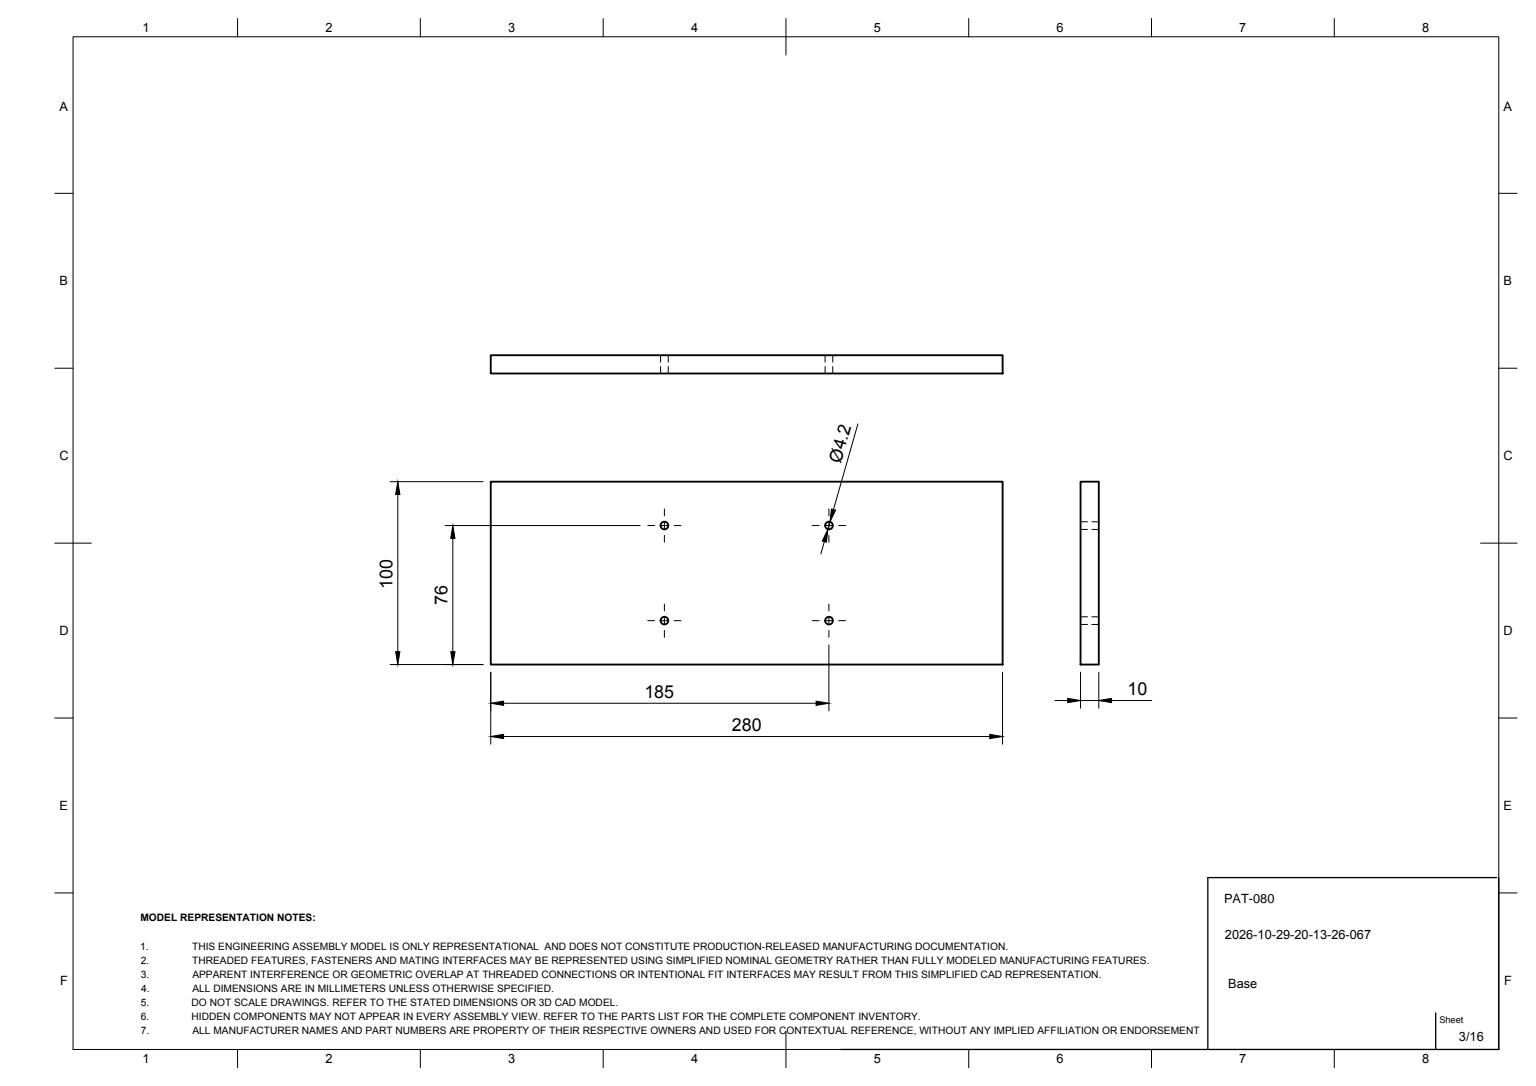
ISO-10303-21;
HEADER;
/* Generated by software containing ST-Developer
 * from STEP Tools, Inc. (www.steptools.com) 
 */

FILE_DESCRIPTION(
/* description */ ('PAT-080'),
/* implementation_level */ '2;1');

FILE_NAME(
/* name */ 'Base.step',
/* time_stamp */ '2026-10-29T20:13:47-07:00',
/* author */ (''),
/* organization */ (''),
/* preprocessor_version */ 'ST-DEVELOPER v20.2',
/* originating_system */ 'Autodesk Translation Framework v15.17.0.0',
/* authorisation */ '');

FILE_SCHEMA (('AUTOMOTIVE_DESIGN { 1 0 10303 214 3 1 1 }'));
ENDSEC;

DATA;
#10=MECHANICAL_DESIGN_GEOMETRIC_PRESENTATION_REPRESENTATION('',(#246),#6878);
#208=SHAPE_REPRESENTATION_RELATIONSHIP('SRR','None',#6964,#227);
#227=ADVANCED_BREP_SHAPE_REPRESENTATION('',(#265),#6859);
#246=STYLED_ITEM('',(#7108),#265);
#265=MANIFOLD_SOLID_BREP('Body1',#3862);
#281=FACE_BOUND('',#735,.T.);
#282=FACE_BOUND('',#736,.T.);
#283=FACE_BOUND('',#737,.T.);
#284=FACE_BOUND('',#738,.T.);
#285=FACE_BOUND('',#740,.T.);
#286=FACE_BOUND('',#741,.T.);
#287=FACE_BOUND('',#742,.T.);
#288=FACE_BOUND('',#743,.T.);
#357=PLANE('',#4108);
#358=PLANE('',#4109);
#359=PLANE('',#4110);
#360=PLANE('',#4111);
#361=PLANE('',#4112);
#362=PLANE('',#4113);
#500=FACE_OUTER_BOUND('',#726,.T.);
#501=FACE_OUTER_BOUND('',#727,.T.);
#502=FACE_OUTER_BOUND('',#728,.T.);
#503=FACE_OUTER_BOUND('',#729,.T.);
#504=FACE_OUTER_BOUND('',#730,.T.);
#505=FACE_OUTER_BOUND('',#731,.T.);
#506=FACE_OUTER_BOUND('',#732,.T.);
#507=FACE_OUTER_BOUND('',#733,.T.);
#508=FACE_OUTER_BOUND('',#734,.T.);
#509=FACE_OUTER_BOUND('',#739,.T.);
#726=EDGE_LOOP('',(#2608,#2609,#2610,#2611));
#727=EDGE_LOOP('',(#2612,#2613,#2614,#2615));
#728=EDGE_LOOP('',(#2616,#2617,#2618,#2619));
#729=EDGE_LOOP('',(#2620,#2621,#2622,#2623));
#730=EDGE_LOOP('',(#2624,#2625,#2626,#2627));
#731=EDGE_LOOP('',(#2628,#2629,#2630,#2631));
#732=EDGE_LOOP('',(#2632,#2633,#2634,#2635));
#733=EDGE_LOOP('',(#2636,#2637,#2638,#2639));
#734=EDGE_LOOP('',(#2640,#2641,#2642,#2643));
#735=EDGE_LOOP('',(#2644));
#736=EDGE_LOOP('',(#2645));
#737=EDGE_LOOP('',(#2646));
#738=EDGE_LOOP('',(#2647));
#739=EDGE_LOOP('',(#2648,#2649,#2650,#2651));
#740=EDGE_LOOP('',(#2652));
#741=EDGE_LOOP('',(#2653));
#742=EDGE_LOOP('',(#2654));
#743=EDGE_LOOP('',(#2655));
#1028=LINE('',#5735,#1343);
#1029=LINE('',#5741,#1344);
#1030=LINE('',#5747,#1345);
#1031=LINE('',#5753,#1346);
#1032=LINE('',#5758,#1347);
#1033=LINE('',#5760,#1348);
#1034=LINE('',#5762,#1349);
#1035=LINE('',#5763,#1350);
#1036=LINE('',#5766,#1351);
#1037=LINE('',#5768,#1352);
#1038=LINE('',#5769,#1353);
#1039=LINE('',#5772,#1354);
#1040=LINE('',#5774,#1355);
#1041=LINE('',#5775,#1356);
#1042=LINE('',#5777,#1357);
#1043=LINE('',#5778,#1358);
#1343=VECTOR('',#4542,0.21);
#1344=VECTOR('',#4549,0.21);
#1345=VECTOR('',#4556,0.21);
#1346=VECTOR('',#4563,0.21);
#1347=VECTOR('',#4568,1.);
#1348=VECTOR('',#4569,1.);
#1349=VECTOR('',#4570,1.);
#1350=VECTOR('',#4571,1.);
#1351=VECTOR('',#4574,1.);
#1352=VECTOR('',#4575,1.);
#1353=VECTOR('',#4576,1.);
#1354=VECTOR('',#4579,1.);
#1355=VECTOR('',#4580,1.);
#1356=VECTOR('',#4581,1.);
#1357=VECTOR('',#4584,1.);
#1358=VECTOR('',#4585,1.);
#1658=CIRCLE('',#4097,0.21);
#1659=CIRCLE('',#4098,0.21);
#1660=CIRCLE('',#4100,0.21);
#1661=CIRCLE('',#4101,0.21);
#1662=CIRCLE('',#4103,0.21);
#1663=CIRCLE('',#4104,0.21);
#1664=CIRCLE('',#4106,0.21);
#1665=CIRCLE('',#4107,0.21);
#1810=VERTEX_POINT('',#5732);
#1811=VERTEX_POINT('',#5734);
#1812=VERTEX_POINT('',#5738);
#1813=VERTEX_POINT('',#5740);
#1814=VERTEX_POINT('',#5744);
#1815=VERTEX_POINT('',#5746);
#1816=VERTEX_POINT('',#5750);
#1817=VERTEX_POINT('',#5752);
#1818=VERTEX_POINT('',#5756);
#1819=VERTEX_POINT('',#5757);
#1820=VERTEX_POINT('',#5759);
#1821=VERTEX_POINT('',#5761);
#1822=VERTEX_POINT('',#5765);
#1823=VERTEX_POINT('',#5767);
#1824=VERTEX_POINT('',#5771);
#1825=VERTEX_POINT('',#5773);
#2127=EDGE_CURVE('',#1810,#1810,#1658,.T.);
#2128=EDGE_CURVE('',#1810,#1811,#1028,.T.);
#2129=EDGE_CURVE('',#1811,#1811,#1659,.T.);
#2130=EDGE_CURVE('',#1812,#1812,#1660,.T.);
#2131=EDGE_CURVE('',#1812,#1813,#1029,.T.);
#2132=EDGE_CURVE('',#1813,#1813,#1661,.T.);
#2133=EDGE_CURVE('',#1814,#1814,#1662,.T.);
#2134=EDGE_CURVE('',#1814,#1815,#1030,.T.);
#2135=EDGE_CURVE('',#1815,#1815,#1663,.T.);
#2136=EDGE_CURVE('',#1816,#1816,#1664,.T.);
#2137=EDGE_CURVE('',#1816,#1817,#1031,.T.);
#2138=EDGE_CURVE('',#1817,#1817,#1665,.T.);
#2139=EDGE_CURVE('',#1818,#1819,#1032,.T.);
#2140=EDGE_CURVE('',#1819,#1820,#1033,.T.);
#2141=EDGE_CURVE('',#1821,#1820,#1034,.T.);
#2142=EDGE_CURVE('',#1818,#1821,#1035,.T.);
#2143=EDGE_CURVE('',#1822,#1818,#1036,.T.);
#2144=EDGE_CURVE('',#1823,#1821,#1037,.T.);
#2145=EDGE_CURVE('',#1822,#1823,#1038,.T.);
#2146=EDGE_CURVE('',#1824,#1822,#1039,.T.);
#2147=EDGE_CURVE('',#1825,#1823,#1040,.T.);
#2148=EDGE_CURVE('',#1824,#1825,#1041,.T.);
#2149=EDGE_CURVE('',#1819,#1824,#1042,.T.);
#2150=EDGE_CURVE('',#1820,#1825,#1043,.T.);
#2608=ORIENTED_EDGE('',*,*,#2127,.F.);
#2609=ORIENTED_EDGE('',*,*,#2128,.T.);
#2610=ORIENTED_EDGE('',*,*,#2129,.F.);
#2611=ORIENTED_EDGE('',*,*,#2128,.F.);
#2612=ORIENTED_EDGE('',*,*,#2130,.F.);
#2613=ORIENTED_EDGE('',*,*,#2131,.T.);
#2614=ORIENTED_EDGE('',*,*,#2132,.F.);
#2615=ORIENTED_EDGE('',*,*,#2131,.F.);
#2616=ORIENTED_EDGE('',*,*,#2133,.F.);
#2617=ORIENTED_EDGE('',*,*,#2134,.T.);
#2618=ORIENTED_EDGE('',*,*,#2135,.F.);
#2619=ORIENTED_EDGE('',*,*,#2134,.F.);
#2620=ORIENTED_EDGE('',*,*,#2136,.F.);
#2621=ORIENTED_EDGE('',*,*,#2137,.T.);
#2622=ORIENTED_EDGE('',*,*,#2138,.F.);
#2623=ORIENTED_EDGE('',*,*,#2137,.F.);
#2624=ORIENTED_EDGE('',*,*,#2139,.T.);
#2625=ORIENTED_EDGE('',*,*,#2140,.T.);
#2626=ORIENTED_EDGE('',*,*,#2141,.F.);
#2627=ORIENTED_EDGE('',*,*,#2142,.F.);
#2628=ORIENTED_EDGE('',*,*,#2143,.T.);
#2629=ORIENTED_EDGE('',*,*,#2142,.T.);
#2630=ORIENTED_EDGE('',*,*,#2144,.F.);
#2631=ORIENTED_EDGE('',*,*,#2145,.F.);
#2632=ORIENTED_EDGE('',*,*,#2146,.T.);
#2633=ORIENTED_EDGE('',*,*,#2145,.T.);
#2634=ORIENTED_EDGE('',*,*,#2147,.F.);
#2635=ORIENTED_EDGE('',*,*,#2148,.F.);
#2636=ORIENTED_EDGE('',*,*,#2149,.T.);
#2637=ORIENTED_EDGE('',*,*,#2148,.T.);
#2638=ORIENTED_EDGE('',*,*,#2150,.F.);
#2639=ORIENTED_EDGE('',*,*,#2140,.F.);
#2640=ORIENTED_EDGE('',*,*,#2150,.T.);
#2641=ORIENTED_EDGE('',*,*,#2147,.T.);
#2642=ORIENTED_EDGE('',*,*,#2144,.T.);
#2643=ORIENTED_EDGE('',*,*,#2141,.T.);
#2644=ORIENTED_EDGE('',*,*,#2129,.T.);
#2645=ORIENTED_EDGE('',*,*,#2132,.T.);
#2646=ORIENTED_EDGE('',*,*,#2135,.T.);
#2647=ORIENTED_EDGE('',*,*,#2138,.T.);
#2648=ORIENTED_EDGE('',*,*,#2149,.F.);
#2649=ORIENTED_EDGE('',*,*,#2139,.F.);
#2650=ORIENTED_EDGE('',*,*,#2143,.F.);
#2651=ORIENTED_EDGE('',*,*,#2146,.F.);
#2652=ORIENTED_EDGE('',*,*,#2127,.T.);
#2653=ORIENTED_EDGE('',*,*,#2130,.T.);
#2654=ORIENTED_EDGE('',*,*,#2133,.T.);
#2655=ORIENTED_EDGE('',*,*,#2136,.T.);
#3570=CYLINDRICAL_SURFACE('',#4096,0.21);
#3571=CYLINDRICAL_SURFACE('',#4099,0.21);
#3572=CYLINDRICAL_SURFACE('',#4102,0.21);
#3573=CYLINDRICAL_SURFACE('',#4105,0.21);
#3636=ADVANCED_FACE('',(#500),#3570,.F.);
#3637=ADVANCED_FACE('',(#501),#3571,.F.);
#3638=ADVANCED_FACE('',(#502),#3572,.F.);
#3639=ADVANCED_FACE('',(#503),#3573,.F.);
#3640=ADVANCED_FACE('',(#504),#357,.T.);
#3641=ADVANCED_FACE('',(#505),#358,.T.);
#3642=ADVANCED_FACE('',(#506),#359,.T.);
#3643=ADVANCED_FACE('',(#507),#360,.T.);
#3644=ADVANCED_FACE('',(#508,#281,#282,#283,#284),#361,.T.);
#3645=ADVANCED_FACE('',(#509,#285,#286,#287,#288),#362,.F.);
#3862=CLOSED_SHELL('',(#3636,#3637,#3638,#3639,#3640,#3641,#3642,#3643,
#3644,#3645));
#4095=AXIS2_PLACEMENT_3D('',#5730,#4536,#4537);
#4096=AXIS2_PLACEMENT_3D('',#5731,#4538,#4539);
#4097=AXIS2_PLACEMENT_3D('',#5733,#4540,#4541);
#4098=AXIS2_PLACEMENT_3D('',#5736,#4543,#4544);
#4099=AXIS2_PLACEMENT_3D('',#5737,#4545,#4546);
#4100=AXIS2_PLACEMENT_3D('',#5739,#4547,#4548);
#4101=AXIS2_PLACEMENT_3D('',#5742,#4550,#4551);
#4102=AXIS2_PLACEMENT_3D('',#5743,#4552,#4553);
#4103=AXIS2_PLACEMENT_3D('',#5745,#4554,#4555);
#4104=AXIS2_PLACEMENT_3D('',#5748,#4557,#4558);
#4105=AXIS2_PLACEMENT_3D('',#5749,#4559,#4560);
#4106=AXIS2_PLACEMENT_3D('',#5751,#4561,#4562);
#4107=AXIS2_PLACEMENT_3D('',#5754,#4564,#4565);
#4108=AXIS2_PLACEMENT_3D('',#5755,#4566,#4567);
#4109=AXIS2_PLACEMENT_3D('',#5764,#4572,#4573);
#4110=AXIS2_PLACEMENT_3D('',#5770,#4577,#4578);
#4111=AXIS2_PLACEMENT_3D('',#5776,#4582,#4583);
#4112=AXIS2_PLACEMENT_3D('',#5779,#4586,#4587);
#4113=AXIS2_PLACEMENT_3D('',#5780,#4588,#4589);
#4536=DIRECTION('axis',(0.,0.,1.));
#4537=DIRECTION('refdir',(1.,0.,0.));
#4538=DIRECTION('center_axis',(0.,0.,1.));
#4539=DIRECTION('ref_axis',(1.,0.,0.));
#4540=DIRECTION('center_axis',(0.,0.,1.));
#4541=DIRECTION('ref_axis',(1.,0.,0.));
#4542=DIRECTION('',(0.,0.,1.));
#4543=DIRECTION('center_axis',(0.,0.,-1.));
#4544=DIRECTION('ref_axis',(1.,0.,0.));
#4545=DIRECTION('center_axis',(0.,0.,1.));
#4546=DIRECTION('ref_axis',(1.,0.,0.));
#4547=DIRECTION('center_axis',(0.,0.,1.));
#4548=DIRECTION('ref_axis',(1.,0.,0.));
#4549=DIRECTION('',(0.,0.,1.));
#4550=DIRECTION('center_axis',(0.,0.,-1.));
#4551=DIRECTION('ref_axis',(1.,0.,0.));
#4552=DIRECTION('center_axis',(0.,0.,1.));
#4553=DIRECTION('ref_axis',(1.,0.,0.));
#4554=DIRECTION('center_axis',(0.,0.,1.));
#4555=DIRECTION('ref_axis',(1.,0.,0.));
#4556=DIRECTION('',(0.,0.,1.));
#4557=DIRECTION('center_axis',(0.,0.,-1.));
#4558=DIRECTION('ref_axis',(1.,0.,0.));
#4559=DIRECTION('center_axis',(0.,0.,1.));
#4560=DIRECTION('ref_axis',(1.,0.,0.));
#4561=DIRECTION('center_axis',(0.,0.,1.));
#4562=DIRECTION('ref_axis',(1.,0.,0.));
#4563=DIRECTION('',(0.,0.,1.));
#4564=DIRECTION('center_axis',(0.,0.,-1.));
#4565=DIRECTION('ref_axis',(1.,0.,0.));
#4566=DIRECTION('center_axis',(0.,1.,0.));
#4567=DIRECTION('ref_axis',(-1.,0.,0.));
#4568=DIRECTION('',(-1.,0.,0.));
#4569=DIRECTION('',(0.,0.,1.));
#4570=DIRECTION('',(-1.,0.,0.));
#4571=DIRECTION('',(0.,0.,1.));
#4572=DIRECTION('center_axis',(1.,0.,0.));
#4573=DIRECTION('ref_axis',(0.,1.,0.));
#4574=DIRECTION('',(0.,1.,0.));
#4575=DIRECTION('',(0.,1.,0.));
#4576=DIRECTION('',(0.,0.,1.));
#4577=DIRECTION('center_axis',(0.,-1.,0.));
#4578=DIRECTION('ref_axis',(1.,0.,0.));
#4579=DIRECTION('',(1.,0.,0.));
#4580=DIRECTION('',(1.,0.,0.));
#4581=DIRECTION('',(0.,0.,1.));
#4582=DIRECTION('center_axis',(-1.,0.,0.));
#4583=DIRECTION('ref_axis',(0.,-1.,0.));
#4584=DIRECTION('',(0.,-1.,0.));
#4585=DIRECTION('',(0.,-1.,0.));
#4586=DIRECTION('center_axis',(0.,0.,1.));
#4587=DIRECTION('ref_axis',(1.,0.,0.));
#4588=DIRECTION('center_axis',(0.,0.,1.));
#4589=DIRECTION('ref_axis',(1.,0.,0.));
#5730=CARTESIAN_POINT('',(0.,0.,0.));
#5731=CARTESIAN_POINT('Origin',(4.5,-2.6,-0.1));
#5732=CARTESIAN_POINT('',(4.29,-2.6,0.));
#5733=CARTESIAN_POINT('Origin',(4.5,-2.6,0.));
#5734=CARTESIAN_POINT('',(4.29,-2.6,1.));
#5735=CARTESIAN_POINT('',(4.29,-2.6,-0.1));
#5736=CARTESIAN_POINT('Origin',(4.5,-2.6,1.));
#5737=CARTESIAN_POINT('Origin',(-4.5,2.6,-0.1));
#5738=CARTESIAN_POINT('',(-4.71,2.6,0.));
#5739=CARTESIAN_POINT('Origin',(-4.5,2.6,0.));
#5740=CARTESIAN_POINT('',(-4.71,2.6,1.));
#5741=CARTESIAN_POINT('',(-4.71,2.6,-0.1));
#5742=CARTESIAN_POINT('Origin',(-4.5,2.6,1.));
#5743=CARTESIAN_POINT('Origin',(-4.5,-2.6,-0.1));
#5744=CARTESIAN_POINT('',(-4.71,-2.6,0.));
#5745=CARTESIAN_POINT('Origin',(-4.5,-2.6,0.));
#5746=CARTESIAN_POINT('',(-4.71,-2.6,1.));
#5747=CARTESIAN_POINT('',(-4.71,-2.6,-0.1));
#5748=CARTESIAN_POINT('Origin',(-4.5,-2.6,1.));
#5749=CARTESIAN_POINT('Origin',(4.5,2.6,-0.1));
#5750=CARTESIAN_POINT('',(4.29,2.6,0.));
#5751=CARTESIAN_POINT('Origin',(4.5,2.6,0.));
#5752=CARTESIAN_POINT('',(4.29,2.6,1.));
#5753=CARTESIAN_POINT('',(4.29,2.6,-0.1));
#5754=CARTESIAN_POINT('Origin',(4.5,2.6,1.));
#5755=CARTESIAN_POINT('Origin',(14.,5.,0.));
#5756=CARTESIAN_POINT('',(14.,5.,0.));
#5757=CARTESIAN_POINT('',(-14.,5.,0.));
#5758=CARTESIAN_POINT('',(14.,5.,0.));
#5759=CARTESIAN_POINT('',(-14.,5.,1.));
#5760=CARTESIAN_POINT('',(-14.,5.,0.));
#5761=CARTESIAN_POINT('',(14.,5.,1.));
#5762=CARTESIAN_POINT('',(14.,5.,1.));
#5763=CARTESIAN_POINT('',(14.,5.,0.));
#5764=CARTESIAN_POINT('Origin',(14.,-5.,0.));
#5765=CARTESIAN_POINT('',(14.,-5.,0.));
#5766=CARTESIAN_POINT('',(14.,-5.,0.));
#5767=CARTESIAN_POINT('',(14.,-5.,1.));
#5768=CARTESIAN_POINT('',(14.,-5.,1.));
#5769=CARTESIAN_POINT('',(14.,-5.,0.));
#5770=CARTESIAN_POINT('Origin',(-14.,-5.,0.));
#5771=CARTESIAN_POINT('',(-14.,-5.,0.));
#5772=CARTESIAN_POINT('',(-14.,-5.,0.));
#5773=CARTESIAN_POINT('',(-14.,-5.,1.));
#5774=CARTESIAN_POINT('',(-14.,-5.,1.));
#5775=CARTESIAN_POINT('',(-14.,-5.,0.));
#5776=CARTESIAN_POINT('Origin',(-14.,5.,0.));
#5777=CARTESIAN_POINT('',(-14.,5.,0.));
#5778=CARTESIAN_POINT('',(-14.,5.,1.));
#5779=CARTESIAN_POINT('Origin',(0.,0.,1.));
#5780=CARTESIAN_POINT('Origin',(0.,0.,0.));
#6838=UNCERTAINTY_MEASURE_WITH_UNIT(LENGTH_MEASURE(0.001),#6879,
'DISTANCE_ACCURACY_VALUE',
'Maximum model space distance between geometric entities at asserted c
onnectivities');
#6857=UNCERTAINTY_MEASURE_WITH_UNIT(LENGTH_MEASURE(0.001),#6879,
'DISTANCE_ACCURACY_VALUE',
'Maximum model space distance between geometric entities at asserted c
onnectivities');
#6859=(
GEOMETRIC_REPRESENTATION_CONTEXT(3)
GLOBAL_UNCERTAINTY_ASSIGNED_CONTEXT((#6838))
GLOBAL_UNIT_ASSIGNED_CONTEXT((#6879,#6881,#6882))
REPRESENTATION_CONTEXT('','3D')
);
#6878=(
GEOMETRIC_REPRESENTATION_CONTEXT(3)
GLOBAL_UNCERTAINTY_ASSIGNED_CONTEXT((#6857))
GLOBAL_UNIT_ASSIGNED_CONTEXT((#6879,#6881,#6882))
REPRESENTATION_CONTEXT('','3D')
);
#6879=(
LENGTH_UNIT()
NAMED_UNIT(*)
SI_UNIT(.CENTI.,.METRE.)
);
#6881=(
NAMED_UNIT(*)
PLANE_ANGLE_UNIT()
SI_UNIT($,.RADIAN.)
);
#6882=(
NAMED_UNIT(*)
SI_UNIT($,.STERADIAN.)
SOLID_ANGLE_UNIT()
);
#6884=SHAPE_DEFINITION_REPRESENTATION(#6904,#6964);
#6904=PRODUCT_DEFINITION_SHAPE('',$,#6985);
#6964=SHAPE_REPRESENTATION('',(#4095),#6859);
#6983=PRODUCT_DEFINITION_CONTEXT('part definition',#7045,'design');
#6985=PRODUCT_DEFINITION('Base','Base',#7005,#6983);
#7005=PRODUCT_DEFINITION_FORMATION('',$,#7048);
#7045=APPLICATION_CONTEXT(
'Core Data for Automotive Mechanical Design Process');
#7046=PRODUCT_CONTEXT('part definition',#7045,'mechanical');
#7048=PRODUCT('Base','Base','Base',(#7046));
#7102=COLOUR_RGB('Dark Blue',0.08,0.2,0.34);
#7103=FILL_AREA_STYLE_COLOUR('',#7102);
#7104=FILL_AREA_STYLE('',(#7103));
#7105=SURFACE_STYLE_FILL_AREA(#7104);
#7106=SURFACE_SIDE_STYLE('',(#7105));
#7107=SURFACE_STYLE_USAGE(.BOTH.,#7106);
#7108=PRESENTATION_STYLE_ASSIGNMENT((#7107));
ENDSEC;
END-ISO-10303-21;
